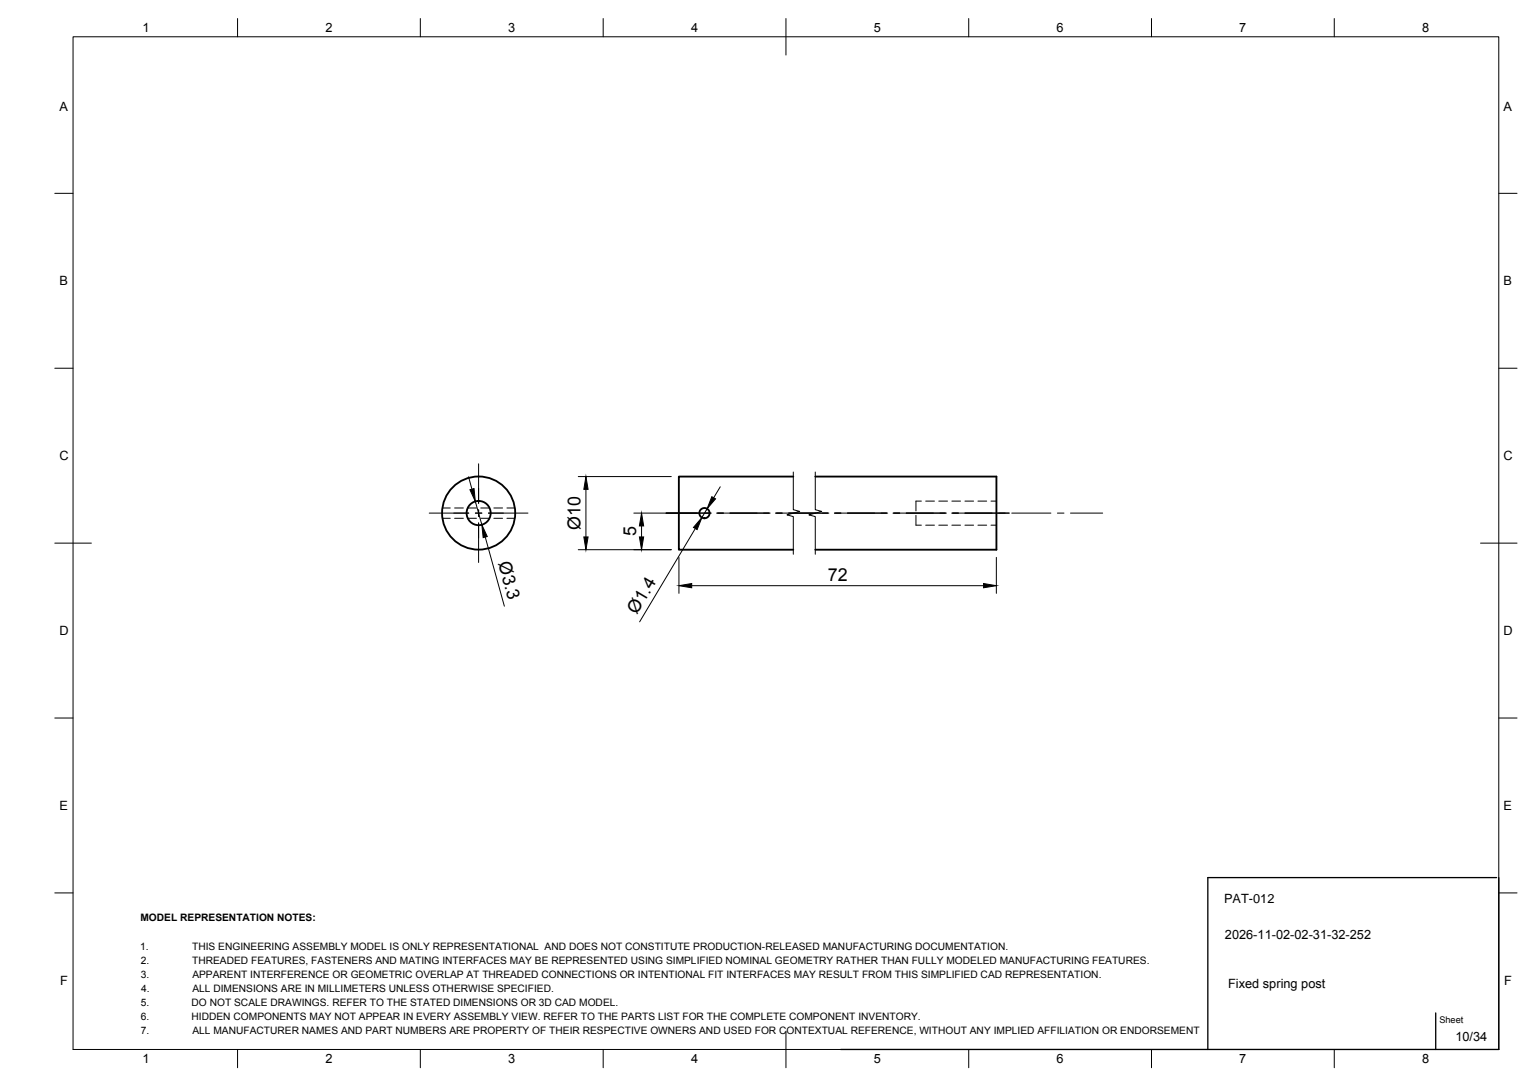
ISO-10303-21;
HEADER;
/* Generated by software containing ST-Developer
 * from STEP Tools, Inc. (www.steptools.com) 
 */

FILE_DESCRIPTION(
/* description */ ('Belt tensioner idler arm'),
/* implementation_level */ '2;1');

FILE_NAME(
/* name */ 'Fixed spring post.step',
/* time_stamp */ '2026-10-28T03:22:15-07:00',
/* author */ (''),
/* organization */ (''),
/* preprocessor_version */ 'ST-DEVELOPER v20.2',
/* originating_system */ 'Autodesk Translation Framework v15.17.0.0',
/* authorisation */ '');

FILE_SCHEMA (('AUTOMOTIVE_DESIGN { 1 0 10303 214 3 1 1 }'));
ENDSEC;

DATA;
#10=MECHANICAL_DESIGN_GEOMETRIC_PRESENTATION_REPRESENTATION('',(#452),#12779);
#322=B_SPLINE_CURVE_WITH_KNOTS('',3,(#9711,#9712,#9713,#9714,#9715,#9716,
#9717,#9718,#9719,#9720,#9721,#9722,#9723,#9724,#9725,#9726,#9727,#9728,
#9729,#9730,#9731,#9732,#9733,#9734,#9735,#9736,#9737,#9738,#9739,#9740,
#9741,#9742,#9743,#9744),.UNSPECIFIED.,.T.,.F.,(4,2,2,2,2,2,2,2,2,2,2,2,
2,2,2,2,4),(0.,0.0264055269244546,0.0528110538489091,0.0792162323581904,
0.105621410867472,0.132026589376753,0.158431767886034,0.184837294810489,
0.211242821734944,0.237648348659398,0.264053875583852,0.290459054093133,
0.316864232602415,0.343269411111696,0.369674589620977,0.396080116545432,
0.422485643469887),.UNSPECIFIED.);
#323=B_SPLINE_CURVE_WITH_KNOTS('',3,(#9747,#9748,#9749,#9750,#9751,#9752,
#9753,#9754,#9755,#9756,#9757,#9758,#9759,#9760,#9761,#9762,#9763,#9764,
#9765,#9766,#9767,#9768,#9769,#9770,#9771,#9772,#9773,#9774,#9775,#9776,
#9777,#9778,#9779,#9780),.UNSPECIFIED.,.T.,.F.,(4,2,2,2,2,2,2,2,2,2,2,2,
2,2,2,2,4),(0.,0.0264055269244546,0.0528110538489091,0.0792162323581904,
0.105621410867472,0.132026589376753,0.158431767886035,0.184837294810489,
0.211242821734943,0.237648348659398,0.264053875583852,0.290459054093133,
0.316864232602415,0.343269411111696,0.369674589620977,0.396080116545432,
0.422485643469887),.UNSPECIFIED.);
#384=SHAPE_REPRESENTATION_RELATIONSHIP('SRR','None',#12930,#418);
#418=ADVANCED_BREP_SHAPE_REPRESENTATION('',(#494),#12747);
#452=STYLED_ITEM('',(#13184),#494);
#494=MANIFOLD_SOLID_BREP('Body1',#6186);
#550=FACE_BOUND('',#1273,.T.);
#551=FACE_BOUND('',#1274,.T.);
#552=FACE_BOUND('',#1277,.T.);
#690=PLANE('',#6685);
#691=PLANE('',#6690);
#692=PLANE('',#6691);
#879=FACE_OUTER_BOUND('',#1269,.T.);
#880=FACE_OUTER_BOUND('',#1270,.T.);
#881=FACE_OUTER_BOUND('',#1271,.T.);
#882=FACE_OUTER_BOUND('',#1272,.T.);
#883=FACE_OUTER_BOUND('',#1275,.T.);
#884=FACE_OUTER_BOUND('',#1276,.T.);
#1269=EDGE_LOOP('',(#4262,#4263,#4264,#4265));
#1270=EDGE_LOOP('',(#4266));
#1271=EDGE_LOOP('',(#4267,#4268,#4269,#4270));
#1272=EDGE_LOOP('',(#4271,#4272,#4273,#4274));
#1273=EDGE_LOOP('',(#4275));
#1274=EDGE_LOOP('',(#4276));
#1275=EDGE_LOOP('',(#4277));
#1276=EDGE_LOOP('',(#4278));
#1277=EDGE_LOOP('',(#4279));
#1760=LINE('',#9706,#2109);
#1761=LINE('',#9746,#2110);
#1762=LINE('',#9785,#2111);
#2109=VECTOR('',#7650,0.165);
#2110=VECTOR('',#7657,0.07);
#2111=VECTOR('',#7662,0.5);
#2435=CIRCLE('',#6683,0.165);
#2436=CIRCLE('',#6684,0.165);
#2437=CIRCLE('',#6688,0.5);
#2438=CIRCLE('',#6689,0.5);
#2828=VERTEX_POINT('',#9703);
#2829=VERTEX_POINT('',#9705);
#2830=VERTEX_POINT('',#9710);
#2831=VERTEX_POINT('',#9745);
#2832=VERTEX_POINT('',#9782);
#2833=VERTEX_POINT('',#9784);
#3386=EDGE_CURVE('',#2828,#2828,#2435,.T.);
#3387=EDGE_CURVE('',#2828,#2829,#1760,.T.);
#3388=EDGE_CURVE('',#2829,#2829,#2436,.T.);
#3389=EDGE_CURVE('',#2830,#2830,#322,.T.);
#3390=EDGE_CURVE('',#2830,#2831,#1761,.T.);
#3391=EDGE_CURVE('',#2831,#2831,#323,.T.);
#3392=EDGE_CURVE('',#2832,#2832,#2437,.T.);
#3393=EDGE_CURVE('',#2832,#2833,#1762,.T.);
#3394=EDGE_CURVE('',#2833,#2833,#2438,.T.);
#4262=ORIENTED_EDGE('',*,*,#3386,.F.);
#4263=ORIENTED_EDGE('',*,*,#3387,.T.);
#4264=ORIENTED_EDGE('',*,*,#3388,.T.);
#4265=ORIENTED_EDGE('',*,*,#3387,.F.);
#4266=ORIENTED_EDGE('',*,*,#3388,.F.);
#4267=ORIENTED_EDGE('',*,*,#3389,.F.);
#4268=ORIENTED_EDGE('',*,*,#3390,.T.);
#4269=ORIENTED_EDGE('',*,*,#3391,.F.);
#4270=ORIENTED_EDGE('',*,*,#3390,.F.);
#4271=ORIENTED_EDGE('',*,*,#3392,.F.);
#4272=ORIENTED_EDGE('',*,*,#3393,.T.);
#4273=ORIENTED_EDGE('',*,*,#3394,.T.);
#4274=ORIENTED_EDGE('',*,*,#3393,.F.);
#4275=ORIENTED_EDGE('',*,*,#3391,.T.);
#4276=ORIENTED_EDGE('',*,*,#3389,.T.);
#4277=ORIENTED_EDGE('',*,*,#3392,.T.);
#4278=ORIENTED_EDGE('',*,*,#3394,.F.);
#4279=ORIENTED_EDGE('',*,*,#3386,.T.);
#5677=CYLINDRICAL_SURFACE('',#6682,0.165);
#5678=CYLINDRICAL_SURFACE('',#6686,0.07);
#5679=CYLINDRICAL_SURFACE('',#6687,0.5);
#5856=ADVANCED_FACE('',(#879),#5677,.F.);
#5857=ADVANCED_FACE('',(#880),#690,.F.);
#5858=ADVANCED_FACE('',(#881),#5678,.F.);
#5859=ADVANCED_FACE('',(#882,#550,#551),#5679,.T.);
#5860=ADVANCED_FACE('',(#883),#691,.T.);
#5861=ADVANCED_FACE('',(#884,#552),#692,.F.);
#6186=CLOSED_SHELL('',(#5856,#5857,#5858,#5859,#5860,#5861));
#6681=AXIS2_PLACEMENT_3D('',#9701,#7644,#7645);
#6682=AXIS2_PLACEMENT_3D('',#9702,#7646,#7647);
#6683=AXIS2_PLACEMENT_3D('',#9704,#7648,#7649);
#6684=AXIS2_PLACEMENT_3D('',#9707,#7651,#7652);
#6685=AXIS2_PLACEMENT_3D('',#9708,#7653,#7654);
#6686=AXIS2_PLACEMENT_3D('',#9709,#7655,#7656);
#6687=AXIS2_PLACEMENT_3D('',#9781,#7658,#7659);
#6688=AXIS2_PLACEMENT_3D('',#9783,#7660,#7661);
#6689=AXIS2_PLACEMENT_3D('',#9786,#7663,#7664);
#6690=AXIS2_PLACEMENT_3D('',#9787,#7665,#7666);
#6691=AXIS2_PLACEMENT_3D('',#9788,#7667,#7668);
#7644=DIRECTION('axis',(0.,0.,1.));
#7645=DIRECTION('refdir',(1.,0.,0.));
#7646=DIRECTION('center_axis',(0.,0.,1.));
#7647=DIRECTION('ref_axis',(1.,0.,0.));
#7648=DIRECTION('center_axis',(0.,0.,1.));
#7649=DIRECTION('ref_axis',(1.,0.,0.));
#7650=DIRECTION('',(0.,0.,1.));
#7651=DIRECTION('center_axis',(0.,0.,1.));
#7652=DIRECTION('ref_axis',(1.,0.,0.));
#7653=DIRECTION('center_axis',(0.,0.,1.));
#7654=DIRECTION('ref_axis',(1.,0.,0.));
#7655=DIRECTION('center_axis',(0.,1.,0.));
#7656=DIRECTION('ref_axis',(1.,0.,0.));
#7657=DIRECTION('',(0.,1.,0.));
#7658=DIRECTION('center_axis',(0.,0.,1.));
#7659=DIRECTION('ref_axis',(1.,0.,0.));
#7660=DIRECTION('center_axis',(0.,0.,1.));
#7661=DIRECTION('ref_axis',(1.,0.,0.));
#7662=DIRECTION('',(0.,0.,-1.));
#7663=DIRECTION('center_axis',(0.,0.,1.));
#7664=DIRECTION('ref_axis',(1.,0.,0.));
#7665=DIRECTION('center_axis',(0.,0.,1.));
#7666=DIRECTION('ref_axis',(1.,0.,0.));
#7667=DIRECTION('center_axis',(0.,0.,1.));
#7668=DIRECTION('ref_axis',(1.,0.,0.));
#9701=CARTESIAN_POINT('',(0.,0.,0.));
#9702=CARTESIAN_POINT('Origin',(0.8,-3.5,-0.1));
#9703=CARTESIAN_POINT('',(0.635,-3.5,0.));
#9704=CARTESIAN_POINT('Origin',(0.8,-3.5,0.));
#9705=CARTESIAN_POINT('',(0.635,-3.5,1.1));
#9706=CARTESIAN_POINT('',(0.635,-3.5,-0.1));
#9707=CARTESIAN_POINT('Origin',(0.8,-3.5,1.1));
#9708=CARTESIAN_POINT('Origin',(0.8,-3.5,1.1));
#9709=CARTESIAN_POINT('Origin',(0.8,-4.1,6.85));
#9710=CARTESIAN_POINT('',(0.73,-3.99507575177946,6.85));
#9711=CARTESIAN_POINT('Ctrl Pts',(0.73,-3.99507575177946,6.85));
#9712=CARTESIAN_POINT('Ctrl Pts',(0.73,-3.99507575177946,6.85880184230815));
#9713=CARTESIAN_POINT('Ctrl Pts',(0.731761420910135,-3.99533471984804,6.86818235803024));
#9714=CARTESIAN_POINT('Ctrl Pts',(0.738908745654556,-3.99626691094106,6.88542542296838));
#9715=CARTESIAN_POINT('Ctrl Pts',(0.744294025343202,-3.99692632385861,6.89328897470932));
#9716=CARTESIAN_POINT('Ctrl Pts',(0.756710943370877,-3.99816160380442,6.90570589273699));
#9717=CARTESIAN_POINT('Ctrl Pts',(0.764574530564745,-3.99881818552376,6.91109123666712));
#9718=CARTESIAN_POINT('Ctrl Pts',(0.781817716198034,-3.99974388505215,6.91823860827541));
#9719=CARTESIAN_POINT('Ctrl Pts',(0.79119827383024,-4.,6.92));
#9720=CARTESIAN_POINT('Ctrl Pts',(0.80880172616976,-4.,6.92));
#9721=CARTESIAN_POINT('Ctrl Pts',(0.818182283801966,-3.99974388505215,6.91823860827541));
#9722=CARTESIAN_POINT('Ctrl Pts',(0.835425469435255,-3.99881818552376,6.91109123666712));
#9723=CARTESIAN_POINT('Ctrl Pts',(0.843289056629123,-3.99816160380442,6.90570589273699));
#9724=CARTESIAN_POINT('Ctrl Pts',(0.855705974656798,-3.99692632385861,6.89328897470932));
#9725=CARTESIAN_POINT('Ctrl Pts',(0.861091254345444,-3.99626691094106,6.88542542296838));
#9726=CARTESIAN_POINT('Ctrl Pts',(0.868238579089865,-3.99533471984804,6.86818235803024));
#9727=CARTESIAN_POINT('Ctrl Pts',(0.87,-3.99507575177946,6.85880184230815));
#9728=CARTESIAN_POINT('Ctrl Pts',(0.87,-3.99507575177946,6.84119815769185));
#9729=CARTESIAN_POINT('Ctrl Pts',(0.868238579089865,-3.99533471984804,6.83181764196976));
#9730=CARTESIAN_POINT('Ctrl Pts',(0.861091254345444,-3.99626691094106,6.81457457703162));
#9731=CARTESIAN_POINT('Ctrl Pts',(0.855705974656798,-3.99692632385861,6.80671102529068));
#9732=CARTESIAN_POINT('Ctrl Pts',(0.843289056629123,-3.99816160380442,6.79429410726301));
#9733=CARTESIAN_POINT('Ctrl Pts',(0.835425469435254,-3.99881818552376,6.78890876333288));
#9734=CARTESIAN_POINT('Ctrl Pts',(0.818182283801966,-3.99974388505215,6.78176139172459));
#9735=CARTESIAN_POINT('Ctrl Pts',(0.808801726169761,-4.,6.78));
#9736=CARTESIAN_POINT('Ctrl Pts',(0.79119827383024,-4.,6.78));
#9737=CARTESIAN_POINT('Ctrl Pts',(0.781817716198034,-3.99974388505215,6.78176139172459));
#9738=CARTESIAN_POINT('Ctrl Pts',(0.764574530564745,-3.99881818552376,6.78890876333288));
#9739=CARTESIAN_POINT('Ctrl Pts',(0.756710943370877,-3.99816160380442,6.79429410726301));
#9740=CARTESIAN_POINT('Ctrl Pts',(0.744294025343202,-3.99692632385861,6.80671102529068));
#9741=CARTESIAN_POINT('Ctrl Pts',(0.738908745654557,-3.99626691094106,6.81457457703162));
#9742=CARTESIAN_POINT('Ctrl Pts',(0.731761420910136,-3.99533471984804,6.83181764196976));
#9743=CARTESIAN_POINT('Ctrl Pts',(0.73,-3.99507575177946,6.84119815769185));
#9744=CARTESIAN_POINT('Ctrl Pts',(0.73,-3.99507575177946,6.85));
#9745=CARTESIAN_POINT('',(0.73,-3.00492424822054,6.85));
#9746=CARTESIAN_POINT('',(0.73,-4.1,6.85));
#9747=CARTESIAN_POINT('Ctrl Pts',(0.73,-3.00492424822054,6.85));
#9748=CARTESIAN_POINT('Ctrl Pts',(0.73,-3.00492424822054,6.84119815769185));
#9749=CARTESIAN_POINT('Ctrl Pts',(0.731761420910135,-3.00466528015196,6.83181764196976));
#9750=CARTESIAN_POINT('Ctrl Pts',(0.738908745654556,-3.00373308905894,6.81457457703162));
#9751=CARTESIAN_POINT('Ctrl Pts',(0.744294025343202,-3.00307367614139,6.80671102529068));
#9752=CARTESIAN_POINT('Ctrl Pts',(0.756710943370877,-3.00183839619558,6.79429410726301));
#9753=CARTESIAN_POINT('Ctrl Pts',(0.764574530564745,-3.00118181447624,6.78890876333288));
#9754=CARTESIAN_POINT('Ctrl Pts',(0.781817716198034,-3.00025611494785,6.78176139172459));
#9755=CARTESIAN_POINT('Ctrl Pts',(0.79119827383024,-3.,6.78));
#9756=CARTESIAN_POINT('Ctrl Pts',(0.808801726169761,-3.,6.78));
#9757=CARTESIAN_POINT('Ctrl Pts',(0.818182283801966,-3.00025611494785,6.78176139172459));
#9758=CARTESIAN_POINT('Ctrl Pts',(0.835425469435254,-3.00118181447624,6.78890876333288));
#9759=CARTESIAN_POINT('Ctrl Pts',(0.843289056629123,-3.00183839619558,6.79429410726301));
#9760=CARTESIAN_POINT('Ctrl Pts',(0.855705974656798,-3.00307367614139,6.80671102529068));
#9761=CARTESIAN_POINT('Ctrl Pts',(0.861091254345444,-3.00373308905894,6.81457457703162));
#9762=CARTESIAN_POINT('Ctrl Pts',(0.868238579089865,-3.00466528015196,6.83181764196976));
#9763=CARTESIAN_POINT('Ctrl Pts',(0.87,-3.00492424822054,6.84119815769185));
#9764=CARTESIAN_POINT('Ctrl Pts',(0.87,-3.00492424822054,6.85880184230815));
#9765=CARTESIAN_POINT('Ctrl Pts',(0.868238579089865,-3.00466528015196,6.86818235803024));
#9766=CARTESIAN_POINT('Ctrl Pts',(0.861091254345444,-3.00373308905894,6.88542542296838));
#9767=CARTESIAN_POINT('Ctrl Pts',(0.855705974656798,-3.00307367614139,6.89328897470932));
#9768=CARTESIAN_POINT('Ctrl Pts',(0.843289056629123,-3.00183839619558,6.90570589273699));
#9769=CARTESIAN_POINT('Ctrl Pts',(0.835425469435255,-3.00118181447624,6.91109123666712));
#9770=CARTESIAN_POINT('Ctrl Pts',(0.818182283801966,-3.00025611494785,6.91823860827541));
#9771=CARTESIAN_POINT('Ctrl Pts',(0.80880172616976,-3.,6.92));
#9772=CARTESIAN_POINT('Ctrl Pts',(0.79119827383024,-3.,6.92));
#9773=CARTESIAN_POINT('Ctrl Pts',(0.781817716198034,-3.00025611494785,6.91823860827541));
#9774=CARTESIAN_POINT('Ctrl Pts',(0.764574530564745,-3.00118181447624,6.91109123666712));
#9775=CARTESIAN_POINT('Ctrl Pts',(0.756710943370877,-3.00183839619558,6.90570589273699));
#9776=CARTESIAN_POINT('Ctrl Pts',(0.744294025343202,-3.00307367614139,6.89328897470932));
#9777=CARTESIAN_POINT('Ctrl Pts',(0.738908745654556,-3.00373308905894,6.88542542296838));
#9778=CARTESIAN_POINT('Ctrl Pts',(0.731761420910135,-3.00466528015196,6.86818235803024));
#9779=CARTESIAN_POINT('Ctrl Pts',(0.73,-3.00492424822054,6.85880184230815));
#9780=CARTESIAN_POINT('Ctrl Pts',(0.73,-3.00492424822054,6.85));
#9781=CARTESIAN_POINT('Origin',(0.8,-3.5,0.));
#9782=CARTESIAN_POINT('',(0.3,-3.5,7.2));
#9783=CARTESIAN_POINT('Origin',(0.8,-3.5,7.2));
#9784=CARTESIAN_POINT('',(0.3,-3.5,0.));
#9785=CARTESIAN_POINT('',(0.3,-3.5,0.));
#9786=CARTESIAN_POINT('Origin',(0.8,-3.5,0.));
#9787=CARTESIAN_POINT('Origin',(0.8,-3.5,7.2));
#9788=CARTESIAN_POINT('Origin',(0.8,-3.5,0.));
#12707=UNCERTAINTY_MEASURE_WITH_UNIT(LENGTH_MEASURE(0.001),#12780,
'DISTANCE_ACCURACY_VALUE',
'Maximum model space distance between geometric entities at asserted c
onnectivities');
#12739=UNCERTAINTY_MEASURE_WITH_UNIT(LENGTH_MEASURE(0.001),#12780,
'DISTANCE_ACCURACY_VALUE',
'Maximum model space distance between geometric entities at asserted c
onnectivities');
#12747=(
GEOMETRIC_REPRESENTATION_CONTEXT(3)
GLOBAL_UNCERTAINTY_ASSIGNED_CONTEXT((#12707))
GLOBAL_UNIT_ASSIGNED_CONTEXT((#12780,#12782,#12783))
REPRESENTATION_CONTEXT('','3D')
);
#12779=(
GEOMETRIC_REPRESENTATION_CONTEXT(3)
GLOBAL_UNCERTAINTY_ASSIGNED_CONTEXT((#12739))
GLOBAL_UNIT_ASSIGNED_CONTEXT((#12780,#12782,#12783))
REPRESENTATION_CONTEXT('','3D')
);
#12780=(
LENGTH_UNIT()
NAMED_UNIT(*)
SI_UNIT(.CENTI.,.METRE.)
);
#12782=(
NAMED_UNIT(*)
PLANE_ANGLE_UNIT()
SI_UNIT($,.RADIAN.)
);
#12783=(
NAMED_UNIT(*)
SI_UNIT($,.STERADIAN.)
SOLID_ANGLE_UNIT()
);
#12791=SHAPE_DEFINITION_REPRESENTATION(#12830,#12930);
#12830=PRODUCT_DEFINITION_SHAPE('',$,#12970);
#12930=SHAPE_REPRESENTATION('',(#6681),#12747);
#12962=PRODUCT_DEFINITION_CONTEXT('part definition',#13081,'design');
#12970=PRODUCT_DEFINITION('Fixed spring post','Fixed spring post',#13009,
#12962);
#13009=PRODUCT_DEFINITION_FORMATION('',$,#13090);
#13081=APPLICATION_CONTEXT(
'Core Data for Automotive Mechanical Design Process');
#13082=PRODUCT_CONTEXT('part definition',#13081,'mechanical');
#13090=PRODUCT('Fixed spring post','Fixed spring post',
'Fixed spring post',(#13082));
#13178=COLOUR_RGB('Grey',0.48,0.52,0.57);
#13179=FILL_AREA_STYLE_COLOUR('',#13178);
#13180=FILL_AREA_STYLE('',(#13179));
#13181=SURFACE_STYLE_FILL_AREA(#13180);
#13182=SURFACE_SIDE_STYLE('',(#13181));
#13183=SURFACE_STYLE_USAGE(.BOTH.,#13182);
#13184=PRESENTATION_STYLE_ASSIGNMENT((#13183));
ENDSEC;
END-ISO-10303-21;
